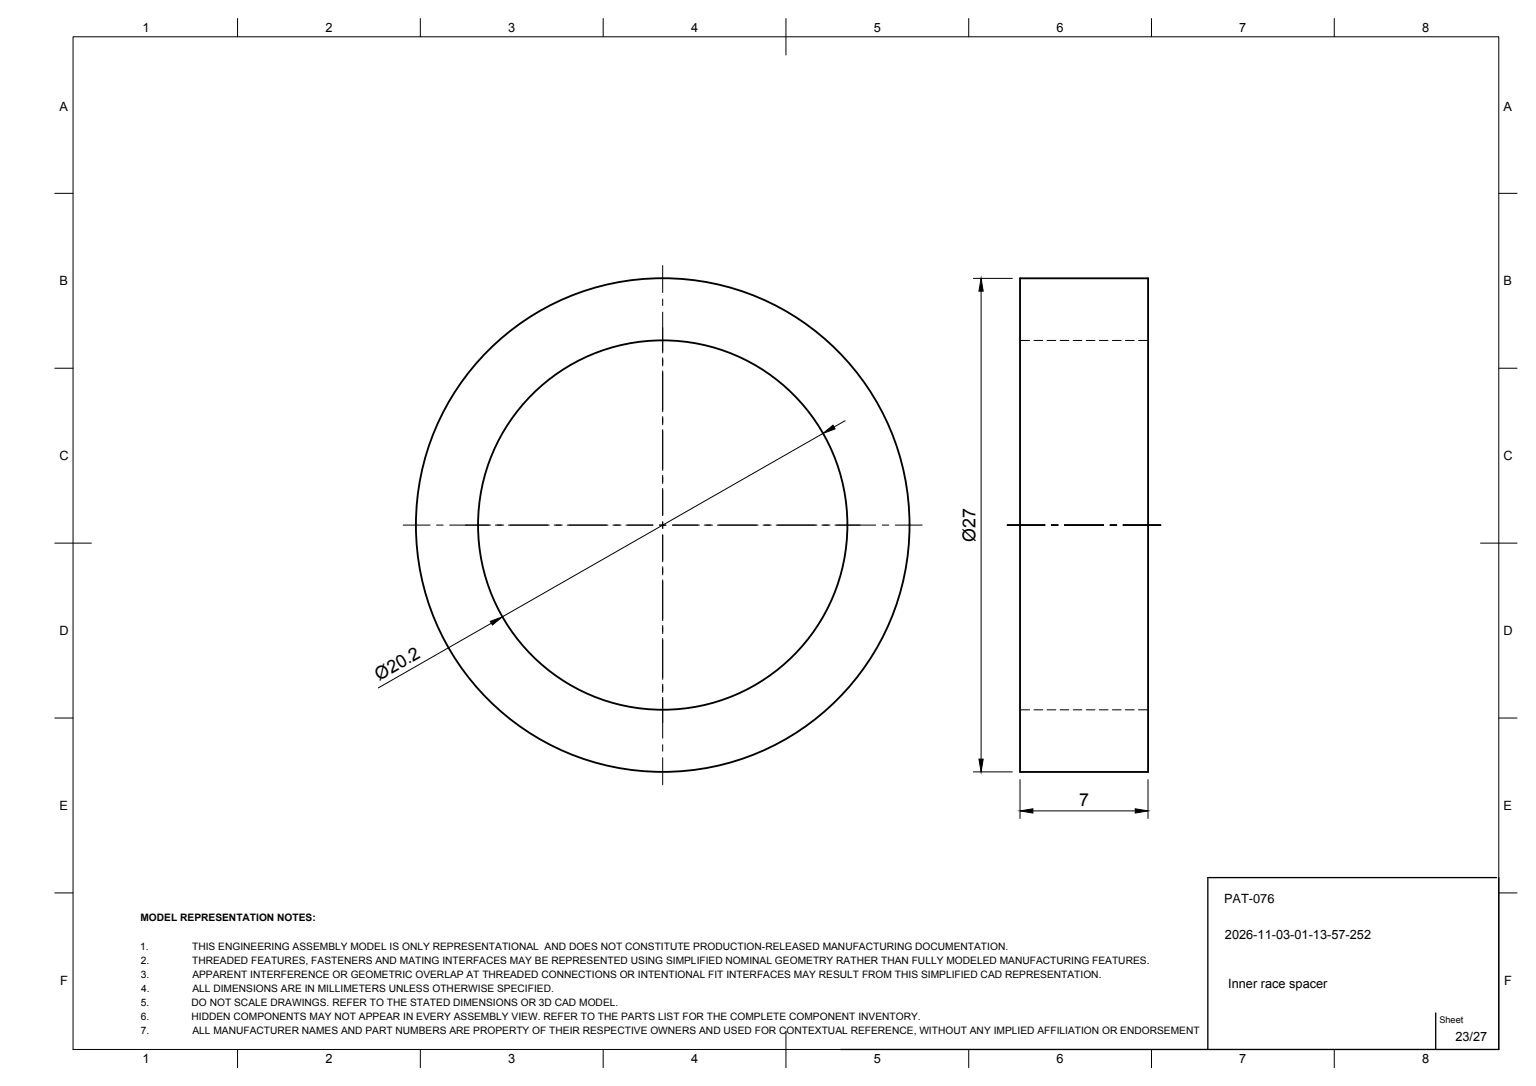
ISO-10303-21;
HEADER;
/* Generated by software containing ST-Developer
 * from STEP Tools, Inc. (www.steptools.com) 
 */

FILE_DESCRIPTION(
/* description */ ('Overhung pulley bearing cartridge'),
/* implementation_level */ '2;1');

FILE_NAME(
/* name */ 'Inner race spacer.step',
/* time_stamp */ '2026-10-28T03:22:33-07:00',
/* author */ (''),
/* organization */ (''),
/* preprocessor_version */ 'ST-DEVELOPER v20.2',
/* originating_system */ 'Autodesk Translation Framework v15.17.0.0',
/* authorisation */ '');

FILE_SCHEMA (('AUTOMOTIVE_DESIGN { 1 0 10303 214 3 1 1 }'));
ENDSEC;

DATA;
#10=MECHANICAL_DESIGN_GEOMETRIC_PRESENTATION_REPRESENTATION('',(#307),#10963);
#255=SHAPE_REPRESENTATION_RELATIONSHIP('SRR','None',#11077,#277);
#277=ADVANCED_BREP_SHAPE_REPRESENTATION('',(#335),#10957);
#307=STYLED_ITEM('',(#11253),#335);
#335=MANIFOLD_SOLID_BREP('Body1',#5676);
#411=FACE_BOUND('',#1172,.T.);
#412=FACE_BOUND('',#1174,.T.);
#540=PLANE('',#6352);
#541=PLANE('',#6353);
#770=FACE_OUTER_BOUND('',#1169,.T.);
#771=FACE_OUTER_BOUND('',#1170,.T.);
#772=FACE_OUTER_BOUND('',#1171,.T.);
#773=FACE_OUTER_BOUND('',#1173,.T.);
#1169=EDGE_LOOP('',(#4423,#4424,#4425,#4426));
#1170=EDGE_LOOP('',(#4427,#4428,#4429,#4430));
#1171=EDGE_LOOP('',(#4431));
#1172=EDGE_LOOP('',(#4432));
#1173=EDGE_LOOP('',(#4433));
#1174=EDGE_LOOP('',(#4434));
#1515=LINE('',#9786,#1857);
#1516=LINE('',#9792,#1858);
#1857=VECTOR('',#7721,1.01);
#1858=VECTOR('',#7728,1.35);
#2192=CIRCLE('',#6347,1.01);
#2193=CIRCLE('',#6348,1.01);
#2194=CIRCLE('',#6350,1.35);
#2195=CIRCLE('',#6351,1.35);
#2645=VERTEX_POINT('',#9783);
#2646=VERTEX_POINT('',#9785);
#2647=VERTEX_POINT('',#9789);
#2648=VERTEX_POINT('',#9791);
#3281=EDGE_CURVE('',#2645,#2645,#2192,.T.);
#3282=EDGE_CURVE('',#2645,#2646,#1515,.T.);
#3283=EDGE_CURVE('',#2646,#2646,#2193,.T.);
#3284=EDGE_CURVE('',#2647,#2647,#2194,.T.);
#3285=EDGE_CURVE('',#2647,#2648,#1516,.T.);
#3286=EDGE_CURVE('',#2648,#2648,#2195,.T.);
#4423=ORIENTED_EDGE('',*,*,#3281,.F.);
#4424=ORIENTED_EDGE('',*,*,#3282,.T.);
#4425=ORIENTED_EDGE('',*,*,#3283,.T.);
#4426=ORIENTED_EDGE('',*,*,#3282,.F.);
#4427=ORIENTED_EDGE('',*,*,#3284,.F.);
#4428=ORIENTED_EDGE('',*,*,#3285,.T.);
#4429=ORIENTED_EDGE('',*,*,#3286,.T.);
#4430=ORIENTED_EDGE('',*,*,#3285,.F.);
#4431=ORIENTED_EDGE('',*,*,#3284,.T.);
#4432=ORIENTED_EDGE('',*,*,#3281,.T.);
#4433=ORIENTED_EDGE('',*,*,#3286,.F.);
#4434=ORIENTED_EDGE('',*,*,#3283,.F.);
#5224=CYLINDRICAL_SURFACE('',#6346,1.01);
#5225=CYLINDRICAL_SURFACE('',#6349,1.35);
#5514=ADVANCED_FACE('',(#770),#5224,.F.);
#5515=ADVANCED_FACE('',(#771),#5225,.T.);
#5516=ADVANCED_FACE('',(#772,#411),#540,.T.);
#5517=ADVANCED_FACE('',(#773,#412),#541,.F.);
#5676=CLOSED_SHELL('',(#5514,#5515,#5516,#5517));
#6345=AXIS2_PLACEMENT_3D('',#9781,#7715,#7716);
#6346=AXIS2_PLACEMENT_3D('',#9782,#7717,#7718);
#6347=AXIS2_PLACEMENT_3D('',#9784,#7719,#7720);
#6348=AXIS2_PLACEMENT_3D('',#9787,#7722,#7723);
#6349=AXIS2_PLACEMENT_3D('',#9788,#7724,#7725);
#6350=AXIS2_PLACEMENT_3D('',#9790,#7726,#7727);
#6351=AXIS2_PLACEMENT_3D('',#9793,#7729,#7730);
#6352=AXIS2_PLACEMENT_3D('',#9794,#7731,#7732);
#6353=AXIS2_PLACEMENT_3D('',#9795,#7733,#7734);
#7715=DIRECTION('axis',(0.,0.,1.));
#7716=DIRECTION('refdir',(1.,0.,0.));
#7717=DIRECTION('center_axis',(0.,1.,0.));
#7718=DIRECTION('ref_axis',(1.,0.,0.));
#7719=DIRECTION('center_axis',(0.,-1.,0.));
#7720=DIRECTION('ref_axis',(1.,0.,0.));
#7721=DIRECTION('',(0.,-1.,0.));
#7722=DIRECTION('center_axis',(0.,-1.,0.));
#7723=DIRECTION('ref_axis',(1.,0.,0.));
#7724=DIRECTION('center_axis',(0.,1.,0.));
#7725=DIRECTION('ref_axis',(1.,0.,0.));
#7726=DIRECTION('center_axis',(0.,1.,0.));
#7727=DIRECTION('ref_axis',(1.,0.,0.));
#7728=DIRECTION('',(0.,-1.,0.));
#7729=DIRECTION('center_axis',(0.,1.,0.));
#7730=DIRECTION('ref_axis',(1.,0.,0.));
#7731=DIRECTION('center_axis',(0.,1.,0.));
#7732=DIRECTION('ref_axis',(1.,0.,0.));
#7733=DIRECTION('center_axis',(0.,1.,0.));
#7734=DIRECTION('ref_axis',(1.,0.,0.));
#9781=CARTESIAN_POINT('',(0.,0.,0.));
#9782=CARTESIAN_POINT('Origin',(0.,5.7,4.5));
#9783=CARTESIAN_POINT('',(-1.01,6.4,4.5));
#9784=CARTESIAN_POINT('Origin',(0.,6.4,4.5));
#9785=CARTESIAN_POINT('',(-1.01,5.7,4.5));
#9786=CARTESIAN_POINT('',(-1.01,5.7,4.5));
#9787=CARTESIAN_POINT('Origin',(0.,5.7,4.5));
#9788=CARTESIAN_POINT('Origin',(0.,5.7,4.5));
#9789=CARTESIAN_POINT('',(-1.35,6.4,4.5));
#9790=CARTESIAN_POINT('Origin',(0.,6.4,4.5));
#9791=CARTESIAN_POINT('',(-1.35,5.7,4.5));
#9792=CARTESIAN_POINT('',(-1.35,5.7,4.5));
#9793=CARTESIAN_POINT('Origin',(0.,5.7,4.5));
#9794=CARTESIAN_POINT('Origin',(0.,6.4,4.5));
#9795=CARTESIAN_POINT('Origin',(0.,5.7,4.5));
#10930=UNCERTAINTY_MEASURE_WITH_UNIT(LENGTH_MEASURE(0.001),#10964,
'DISTANCE_ACCURACY_VALUE',
'Maximum model space distance between geometric entities at asserted c
onnectivities');
#10936=UNCERTAINTY_MEASURE_WITH_UNIT(LENGTH_MEASURE(0.001),#10964,
'DISTANCE_ACCURACY_VALUE',
'Maximum model space distance between geometric entities at asserted c
onnectivities');
#10957=(
GEOMETRIC_REPRESENTATION_CONTEXT(3)
GLOBAL_UNCERTAINTY_ASSIGNED_CONTEXT((#10930))
GLOBAL_UNIT_ASSIGNED_CONTEXT((#10964,#10966,#10967))
REPRESENTATION_CONTEXT('','3D')
);
#10963=(
GEOMETRIC_REPRESENTATION_CONTEXT(3)
GLOBAL_UNCERTAINTY_ASSIGNED_CONTEXT((#10936))
GLOBAL_UNIT_ASSIGNED_CONTEXT((#10964,#10966,#10967))
REPRESENTATION_CONTEXT('','3D')
);
#10964=(
LENGTH_UNIT()
NAMED_UNIT(*)
SI_UNIT(.CENTI.,.METRE.)
);
#10966=(
NAMED_UNIT(*)
PLANE_ANGLE_UNIT()
SI_UNIT($,.RADIAN.)
);
#10967=(
NAMED_UNIT(*)
SI_UNIT($,.STERADIAN.)
SOLID_ANGLE_UNIT()
);
#10988=SHAPE_DEFINITION_REPRESENTATION(#11041,#11077);
#11041=PRODUCT_DEFINITION_SHAPE('',$,#11104);
#11077=SHAPE_REPRESENTATION('',(#6345),#10957);
#11083=PRODUCT_DEFINITION_CONTEXT('part definition',#11163,'design');
#11104=PRODUCT_DEFINITION('Inner race spacer','Inner race spacer',#11130,
#11083);
#11130=PRODUCT_DEFINITION_FORMATION('',$,#11185);
#11163=APPLICATION_CONTEXT(
'Core Data for Automotive Mechanical Design Process');
#11164=PRODUCT_CONTEXT('part definition',#11163,'mechanical');
#11185=PRODUCT('Inner race spacer','Inner race spacer',
'Inner race spacer',(#11164));
#11247=COLOUR_RGB('Grey',0.48,0.52,0.57);
#11248=FILL_AREA_STYLE_COLOUR('',#11247);
#11249=FILL_AREA_STYLE('',(#11248));
#11250=SURFACE_STYLE_FILL_AREA(#11249);
#11251=SURFACE_SIDE_STYLE('',(#11250));
#11252=SURFACE_STYLE_USAGE(.BOTH.,#11251);
#11253=PRESENTATION_STYLE_ASSIGNMENT((#11252));
ENDSEC;
END-ISO-10303-21;
